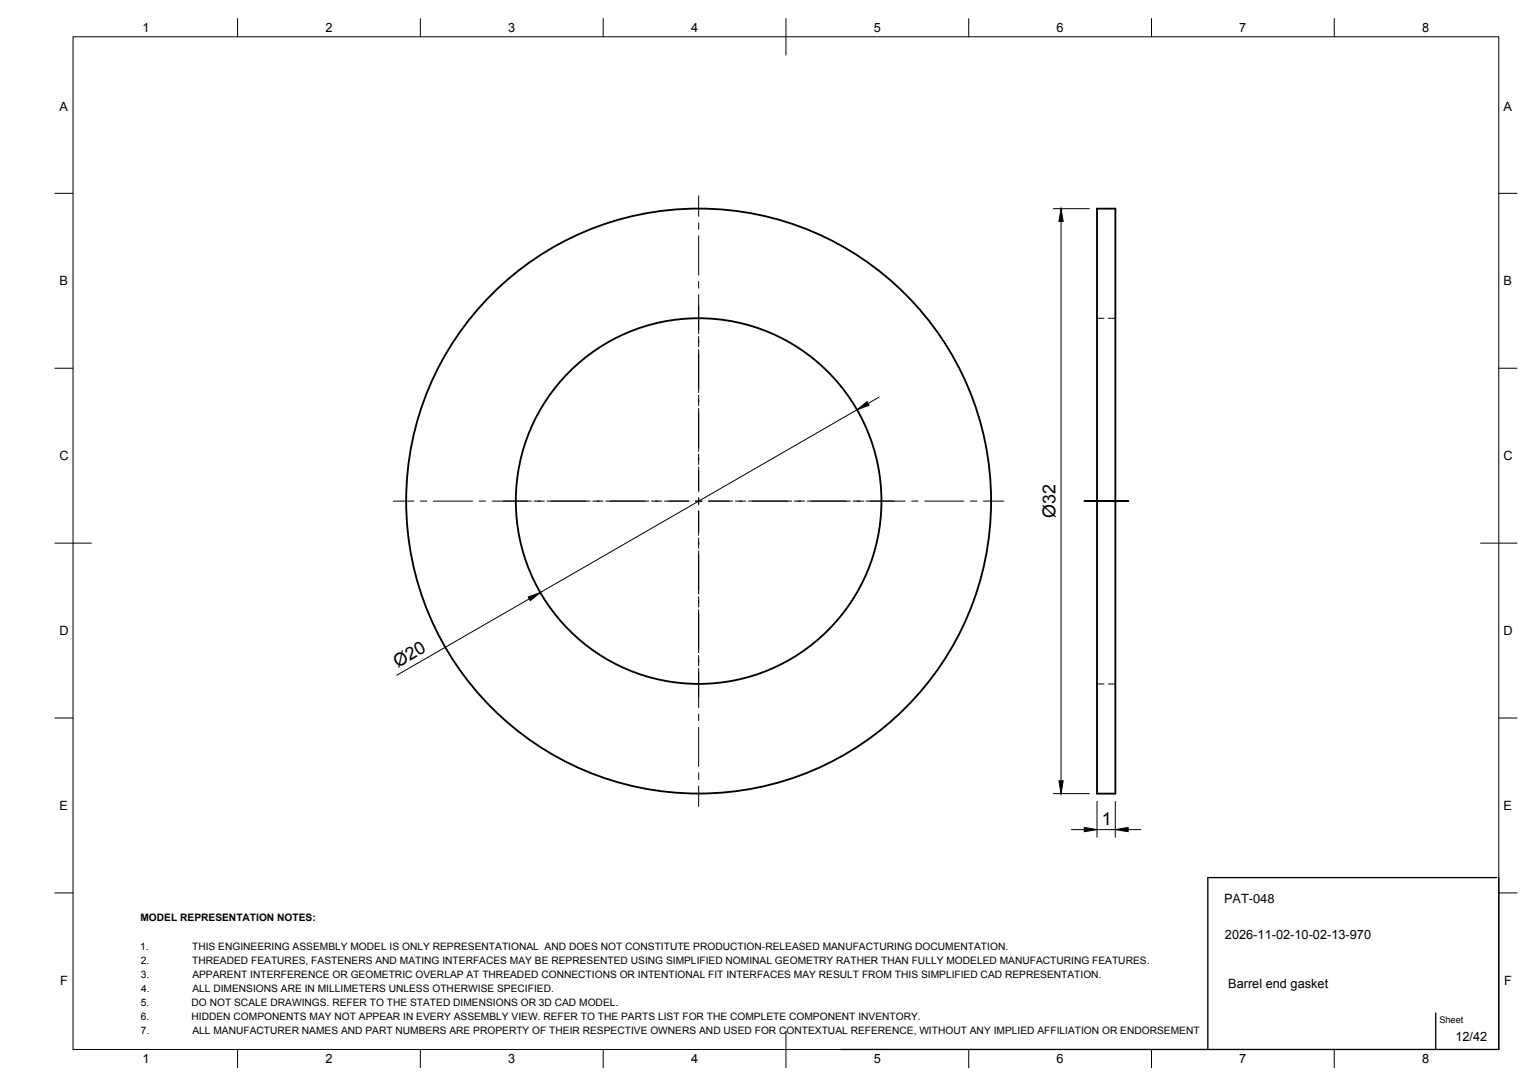
ISO-10303-21;
HEADER;
/* Generated by software containing ST-Developer
 * from STEP Tools, Inc. (www.steptools.com) 
 */

FILE_DESCRIPTION(
/* description */ ('Guided pneumatic stop gate'),
/* implementation_level */ '2;1');

FILE_NAME(
/* name */ 'Barrel end gasket.step',
/* time_stamp */ '2026-10-27T21:43:45-07:00',
/* author */ (''),
/* organization */ (''),
/* preprocessor_version */ 'ST-DEVELOPER v20.2',
/* originating_system */ 'Autodesk Translation Framework v15.17.0.0',
/* authorisation */ '');

FILE_SCHEMA (('AUTOMOTIVE_DESIGN { 1 0 10303 214 3 1 1 }'));
ENDSEC;

DATA;
#10=MECHANICAL_DESIGN_GEOMETRIC_PRESENTATION_REPRESENTATION('',(#542),#14392);
#458=SHAPE_REPRESENTATION_RELATIONSHIP('SRR','None',#14592,#500);
#500=ADVANCED_BREP_SHAPE_REPRESENTATION('',(#584),#14354);
#542=STYLED_ITEM('',(#14884),#584);
#584=MANIFOLD_SOLID_BREP('Body1',#7882);
#665=FACE_BOUND('',#1783,.T.);
#666=FACE_BOUND('',#1785,.T.);
#923=PLANE('',#8651);
#924=PLANE('',#8652);
#1255=FACE_OUTER_BOUND('',#1780,.T.);
#1256=FACE_OUTER_BOUND('',#1781,.T.);
#1257=FACE_OUTER_BOUND('',#1782,.T.);
#1258=FACE_OUTER_BOUND('',#1784,.T.);
#1780=EDGE_LOOP('',(#5874,#5875,#5876,#5877));
#1781=EDGE_LOOP('',(#5878,#5879,#5880,#5881));
#1782=EDGE_LOOP('',(#5882));
#1783=EDGE_LOOP('',(#5883));
#1784=EDGE_LOOP('',(#5884));
#1785=EDGE_LOOP('',(#5885));
#2443=LINE('',#12524,#2988);
#2444=LINE('',#12530,#2989);
#2988=VECTOR('',#10072,1.);
#2989=VECTOR('',#10079,1.6);
#3468=CIRCLE('',#8646,1.);
#3469=CIRCLE('',#8647,1.);
#3470=CIRCLE('',#8649,1.6);
#3471=CIRCLE('',#8650,1.6);
#3911=VERTEX_POINT('',#12521);
#3912=VERTEX_POINT('',#12523);
#3913=VERTEX_POINT('',#12527);
#3914=VERTEX_POINT('',#12529);
#4635=EDGE_CURVE('',#3911,#3911,#3468,.T.);
#4636=EDGE_CURVE('',#3911,#3912,#2443,.T.);
#4637=EDGE_CURVE('',#3912,#3912,#3469,.T.);
#4638=EDGE_CURVE('',#3913,#3913,#3470,.T.);
#4639=EDGE_CURVE('',#3913,#3914,#2444,.T.);
#4640=EDGE_CURVE('',#3914,#3914,#3471,.T.);
#5874=ORIENTED_EDGE('',*,*,#4635,.F.);
#5875=ORIENTED_EDGE('',*,*,#4636,.T.);
#5876=ORIENTED_EDGE('',*,*,#4637,.T.);
#5877=ORIENTED_EDGE('',*,*,#4636,.F.);
#5878=ORIENTED_EDGE('',*,*,#4638,.F.);
#5879=ORIENTED_EDGE('',*,*,#4639,.T.);
#5880=ORIENTED_EDGE('',*,*,#4640,.T.);
#5881=ORIENTED_EDGE('',*,*,#4639,.F.);
#5882=ORIENTED_EDGE('',*,*,#4638,.T.);
#5883=ORIENTED_EDGE('',*,*,#4635,.T.);
#5884=ORIENTED_EDGE('',*,*,#4640,.F.);
#5885=ORIENTED_EDGE('',*,*,#4637,.F.);
#7285=CYLINDRICAL_SURFACE('',#8645,1.);
#7286=CYLINDRICAL_SURFACE('',#8648,1.6);
#7537=ADVANCED_FACE('',(#1255),#7285,.F.);
#7538=ADVANCED_FACE('',(#1256),#7286,.T.);
#7539=ADVANCED_FACE('',(#1257,#665),#923,.T.);
#7540=ADVANCED_FACE('',(#1258,#666),#924,.F.);
#7882=CLOSED_SHELL('',(#7537,#7538,#7539,#7540));
#8644=AXIS2_PLACEMENT_3D('',#12519,#10066,#10067);
#8645=AXIS2_PLACEMENT_3D('',#12520,#10068,#10069);
#8646=AXIS2_PLACEMENT_3D('',#12522,#10070,#10071);
#8647=AXIS2_PLACEMENT_3D('',#12525,#10073,#10074);
#8648=AXIS2_PLACEMENT_3D('',#12526,#10075,#10076);
#8649=AXIS2_PLACEMENT_3D('',#12528,#10077,#10078);
#8650=AXIS2_PLACEMENT_3D('',#12531,#10080,#10081);
#8651=AXIS2_PLACEMENT_3D('',#12532,#10082,#10083);
#8652=AXIS2_PLACEMENT_3D('',#12533,#10084,#10085);
#10066=DIRECTION('axis',(0.,0.,1.));
#10067=DIRECTION('refdir',(1.,0.,0.));
#10068=DIRECTION('center_axis',(0.,1.,0.));
#10069=DIRECTION('ref_axis',(1.,0.,0.));
#10070=DIRECTION('center_axis',(0.,-1.,0.));
#10071=DIRECTION('ref_axis',(1.,0.,0.));
#10072=DIRECTION('',(0.,-1.,0.));
#10073=DIRECTION('center_axis',(0.,-1.,0.));
#10074=DIRECTION('ref_axis',(1.,0.,0.));
#10075=DIRECTION('center_axis',(0.,1.,0.));
#10076=DIRECTION('ref_axis',(1.,0.,0.));
#10077=DIRECTION('center_axis',(0.,1.,0.));
#10078=DIRECTION('ref_axis',(1.,0.,0.));
#10079=DIRECTION('',(0.,-1.,0.));
#10080=DIRECTION('center_axis',(0.,1.,0.));
#10081=DIRECTION('ref_axis',(1.,0.,0.));
#10082=DIRECTION('center_axis',(0.,1.,0.));
#10083=DIRECTION('ref_axis',(1.,0.,0.));
#10084=DIRECTION('center_axis',(0.,1.,0.));
#10085=DIRECTION('ref_axis',(1.,0.,0.));
#12519=CARTESIAN_POINT('',(0.,0.,0.));
#12520=CARTESIAN_POINT('Origin',(0.,1.7,4.5));
#12521=CARTESIAN_POINT('',(-1.,1.8,4.5));
#12522=CARTESIAN_POINT('Origin',(0.,1.8,4.5));
#12523=CARTESIAN_POINT('',(-1.,1.7,4.5));
#12524=CARTESIAN_POINT('',(-1.,1.7,4.5));
#12525=CARTESIAN_POINT('Origin',(0.,1.7,4.5));
#12526=CARTESIAN_POINT('Origin',(0.,1.7,4.5));
#12527=CARTESIAN_POINT('',(-1.6,1.8,4.5));
#12528=CARTESIAN_POINT('Origin',(0.,1.8,4.5));
#12529=CARTESIAN_POINT('',(-1.6,1.7,4.5));
#12530=CARTESIAN_POINT('',(-1.6,1.7,4.5));
#12531=CARTESIAN_POINT('Origin',(0.,1.7,4.5));
#12532=CARTESIAN_POINT('Origin',(0.,1.8,4.5));
#12533=CARTESIAN_POINT('Origin',(0.,1.7,4.5));
#14306=UNCERTAINTY_MEASURE_WITH_UNIT(LENGTH_MEASURE(0.001),#14393,
'DISTANCE_ACCURACY_VALUE',
'Maximum model space distance between geometric entities at asserted c
onnectivities');
#14344=UNCERTAINTY_MEASURE_WITH_UNIT(LENGTH_MEASURE(0.001),#14393,
'DISTANCE_ACCURACY_VALUE',
'Maximum model space distance between geometric entities at asserted c
onnectivities');
#14354=(
GEOMETRIC_REPRESENTATION_CONTEXT(3)
GLOBAL_UNCERTAINTY_ASSIGNED_CONTEXT((#14306))
GLOBAL_UNIT_ASSIGNED_CONTEXT((#14393,#14395,#14396))
REPRESENTATION_CONTEXT('','3D')
);
#14392=(
GEOMETRIC_REPRESENTATION_CONTEXT(3)
GLOBAL_UNCERTAINTY_ASSIGNED_CONTEXT((#14344))
GLOBAL_UNIT_ASSIGNED_CONTEXT((#14393,#14395,#14396))
REPRESENTATION_CONTEXT('','3D')
);
#14393=(
LENGTH_UNIT()
NAMED_UNIT(*)
SI_UNIT(.CENTI.,.METRE.)
);
#14395=(
NAMED_UNIT(*)
PLANE_ANGLE_UNIT()
SI_UNIT($,.RADIAN.)
);
#14396=(
NAMED_UNIT(*)
SI_UNIT($,.STERADIAN.)
SOLID_ANGLE_UNIT()
);
#14406=SHAPE_DEFINITION_REPRESENTATION(#14453,#14592);
#14453=PRODUCT_DEFINITION_SHAPE('',$,#14640);
#14592=SHAPE_REPRESENTATION('',(#8644),#14354);
#14630=PRODUCT_DEFINITION_CONTEXT('part definition',#14773,'design');
#14640=PRODUCT_DEFINITION('Barrel end gasket','Barrel end gasket',#14687,
#14630);
#14687=PRODUCT_DEFINITION_FORMATION('',$,#14784);
#14773=APPLICATION_CONTEXT(
'Core Data for Automotive Mechanical Design Process');
#14774=PRODUCT_CONTEXT('part definition',#14773,'mechanical');
#14784=PRODUCT('Barrel end gasket','Barrel end gasket',
'Barrel end gasket',(#14774));
#14878=COLOUR_RGB('Sky Blue',0.24,0.69,0.87);
#14879=FILL_AREA_STYLE_COLOUR('',#14878);
#14880=FILL_AREA_STYLE('',(#14879));
#14881=SURFACE_STYLE_FILL_AREA(#14880);
#14882=SURFACE_SIDE_STYLE('',(#14881));
#14883=SURFACE_STYLE_USAGE(.BOTH.,#14882);
#14884=PRESENTATION_STYLE_ASSIGNMENT((#14883));
ENDSEC;
END-ISO-10303-21;
